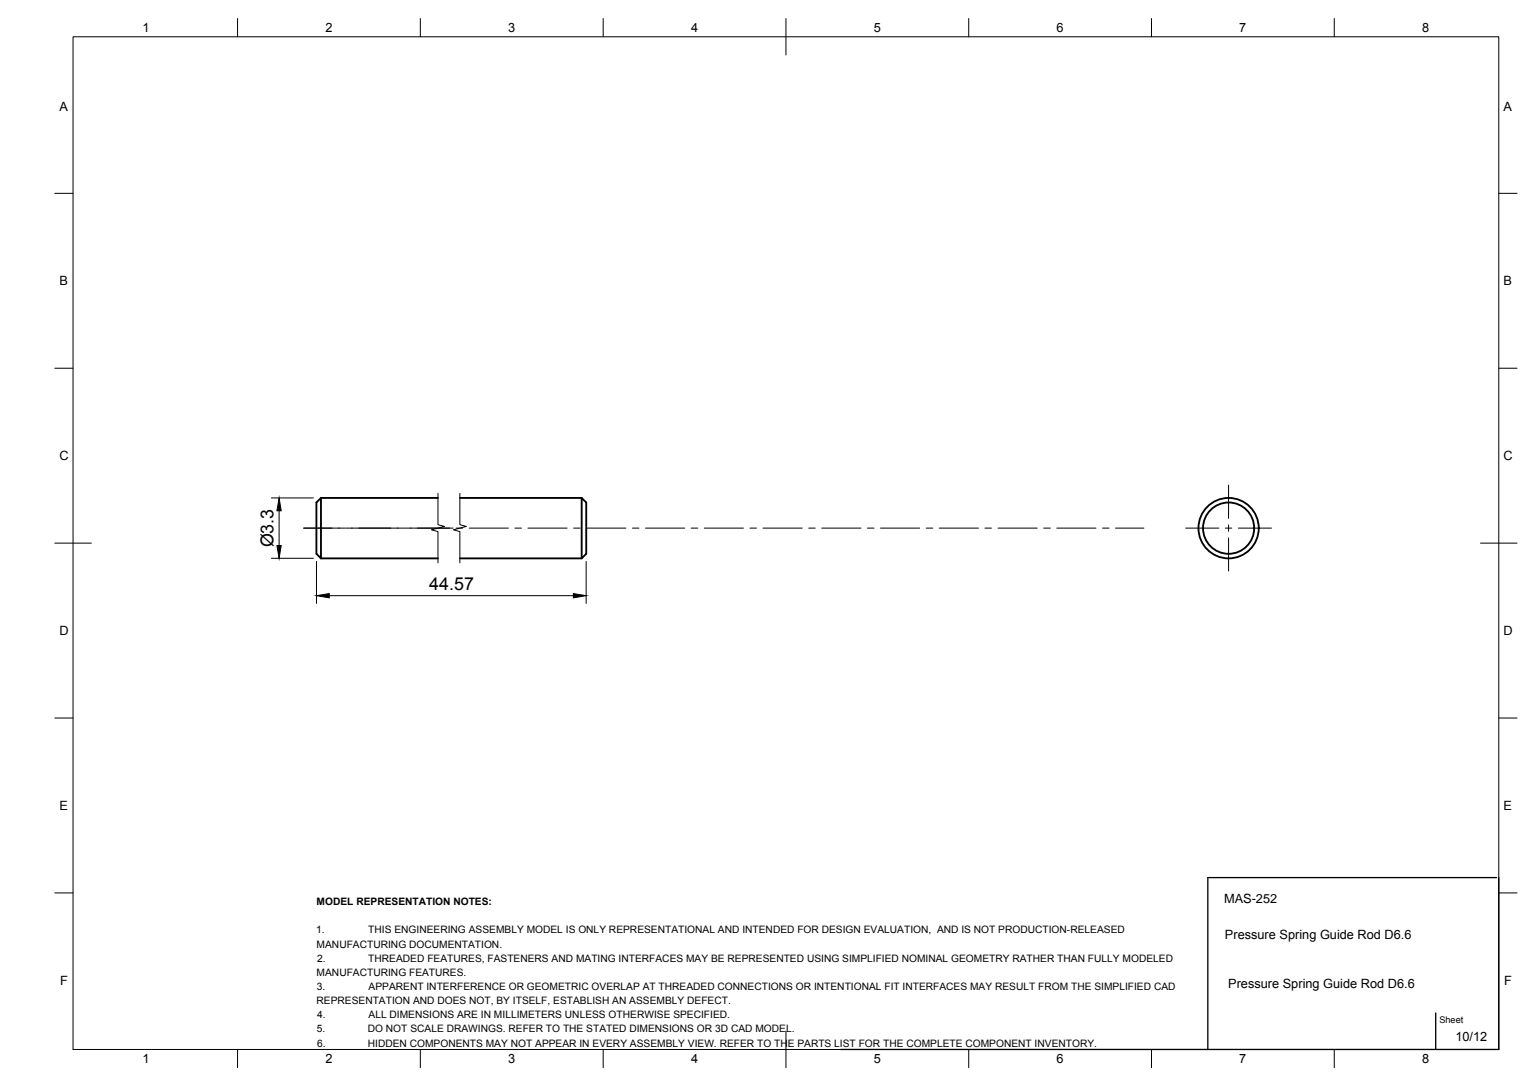
ISO-10303-21;
HEADER;
FILE_DESCRIPTION((''),'2;1');
FILE_NAME('Pressure Spring Guide Rod D6.6.step','2026-10-06T07:01:46+05:00',(''),(''),'','','');
FILE_SCHEMA (('AUTOMOTIVE_DESIGN { 1 0 10303 214 3 1 1 }'));
ENDSEC;
DATA;
#10=MECHANICAL_DESIGN_GEOMETRIC_PRESENTATION_REPRESENTATION('',(#143),#11396);
#99=CONICAL_SURFACE('',#6246,1.525,0.78539816339745) ;
#100=CONICAL_SURFACE('',#6250,1.525,0.78539816339745) ;
#113=SHAPE_REPRESENTATION_RELATIONSHIP('SRR','None',#11460,#128) ;
#128=ADVANCED_BREP_SHAPE_REPRESENTATION('',(#158),#11386) ;
#143=STYLED_ITEM('',(#11544),#158) ;
#158=MANIFOLD_SOLID_BREP('Pressure Spring Guide Rod D6.6',#5574) ;
#466=PLANE('',#6244) ;
#467=PLANE('',#6252) ;
#766=FACE_OUTER_BOUND('',#1130,.T.) ;
#767=FACE_OUTER_BOUND('',#1131,.T.) ;
#768=FACE_OUTER_BOUND('',#1132,.T.) ;
#769=FACE_OUTER_BOUND('',#1133,.T.) ;
#770=FACE_OUTER_BOUND('',#1134,.T.) ;
#1130=EDGE_LOOP('',(#4752)) ;
#1131=EDGE_LOOP('',(#4753,#4754,#4755,#4756)) ;
#1132=EDGE_LOOP('',(#4757,#4758,#4759,#4760)) ;
#1133=EDGE_LOOP('',(#4761,#4762,#4763,#4764)) ;
#1134=EDGE_LOOP('',(#4765)) ;
#1503=LINE('',#10850,#1886) ;
#1504=LINE('',#10854,#1887) ;
#1505=LINE('',#10858,#1888) ;
#1886=VECTOR('',#7693,1.525) ;
#1887=VECTOR('',#7698,1.65) ;
#1888=VECTOR('',#7703,1.525) ;
#2206=CIRCLE('',#6245,1.4) ;
#2207=CIRCLE('',#6247,1.65) ;
#2208=CIRCLE('',#6249,1.65) ;
#2209=CIRCLE('',#6251,1.4) ;
#2635=VERTEX_POINT('',#10845) ;
#2636=VERTEX_POINT('',#10848) ;
#2637=VERTEX_POINT('',#10852) ;
#2638=VERTEX_POINT('',#10856) ;
#3358=EDGE_CURVE('',#2635,#2635,#2206,.T.) ;
#3359=EDGE_CURVE('',#2636,#2636,#2207,.T.) ;
#3360=EDGE_CURVE('',#2636,#2635,#1503,.T.) ;
#3361=EDGE_CURVE('',#2637,#2637,#2208,.T.) ;
#3362=EDGE_CURVE('',#2637,#2636,#1504,.T.) ;
#3363=EDGE_CURVE('',#2638,#2638,#2209,.T.) ;
#3364=EDGE_CURVE('',#2638,#2637,#1505,.T.) ;
#4752=ORIENTED_EDGE('',*,*,#3358,.F.) ;
#4753=ORIENTED_EDGE('',*,*,#3359,.F.) ;
#4754=ORIENTED_EDGE('',*,*,#3360,.T.) ;
#4755=ORIENTED_EDGE('',*,*,#3358,.T.) ;
#4756=ORIENTED_EDGE('',*,*,#3360,.F.) ;
#4757=ORIENTED_EDGE('',*,*,#3361,.F.) ;
#4758=ORIENTED_EDGE('',*,*,#3362,.T.) ;
#4759=ORIENTED_EDGE('',*,*,#3359,.T.) ;
#4760=ORIENTED_EDGE('',*,*,#3362,.F.) ;
#4761=ORIENTED_EDGE('',*,*,#3363,.F.) ;
#4762=ORIENTED_EDGE('',*,*,#3364,.T.) ;
#4763=ORIENTED_EDGE('',*,*,#3361,.T.) ;
#4764=ORIENTED_EDGE('',*,*,#3364,.F.) ;
#4765=ORIENTED_EDGE('',*,*,#3363,.T.) ;
#5208=CYLINDRICAL_SURFACE('',#6248,1.65) ;
#5491=ADVANCED_FACE('',(#766),#466,.T.) ;
#5492=ADVANCED_FACE('',(#767),#99,.T.) ;
#5493=ADVANCED_FACE('',(#768),#5208,.T.) ;
#5494=ADVANCED_FACE('',(#769),#100,.T.) ;
#5495=ADVANCED_FACE('',(#770),#467,.T.) ;
#5574=CLOSED_SHELL('',(#5491,#5492,#5493,#5494,#5495)) ;
#6243=AXIS2_PLACEMENT_3D('',#10843,#7683,#7684) ;
#6244=AXIS2_PLACEMENT_3D('',#10844,#7685,#7686) ;
#6245=AXIS2_PLACEMENT_3D('',#10846,#7687,#7688) ;
#6246=AXIS2_PLACEMENT_3D('',#10847,#7689,#7690) ;
#6247=AXIS2_PLACEMENT_3D('',#10849,#7691,#7692) ;
#6248=AXIS2_PLACEMENT_3D('',#10851,#7694,#7695) ;
#6249=AXIS2_PLACEMENT_3D('',#10853,#7696,#7697) ;
#6250=AXIS2_PLACEMENT_3D('',#10855,#7699,#7700) ;
#6251=AXIS2_PLACEMENT_3D('',#10857,#7701,#7702) ;
#6252=AXIS2_PLACEMENT_3D('',#10859,#7704,#7705) ;
#7683=DIRECTION('axis',(0.,0.,1.)) ;
#7684=DIRECTION('refdir',(1.,0.,0.)) ;
#7685=DIRECTION('center_axis',(0.,0.,-1.)) ;
#7686=DIRECTION('ref_axis',(-1.,0.,0.)) ;
#7687=DIRECTION('center_axis',(0.,0.,1.)) ;
#7688=DIRECTION('ref_axis',(1.,0.,0.)) ;
#7689=DIRECTION('center_axis',(0.,0.,1.)) ;
#7690=DIRECTION('ref_axis',(1.,0.,0.)) ;
#7691=DIRECTION('center_axis',(0.,0.,1.)) ;
#7692=DIRECTION('ref_axis',(1.,0.,0.)) ;
#7693=DIRECTION('',(0.707106781186549,8.65956056235495E-17,-0.707106781186546)) ;
#7694=DIRECTION('center_axis',(0.,0.,1.)) ;
#7695=DIRECTION('ref_axis',(1.,0.,0.)) ;
#7696=DIRECTION('center_axis',(0.,0.,1.)) ;
#7697=DIRECTION('ref_axis',(1.,0.,0.)) ;
#7698=DIRECTION('',(0.,0.,-1.)) ;
#7699=DIRECTION('center_axis',(0.,0.,-1.)) ;
#7700=DIRECTION('ref_axis',(1.,0.,0.)) ;
#7701=DIRECTION('center_axis',(0.,0.,1.)) ;
#7702=DIRECTION('ref_axis',(1.,0.,0.)) ;
#7703=DIRECTION('',(-0.707106781186549,-8.65956056235495E-17,-0.707106781186546)) ;
#7704=DIRECTION('center_axis',(0.,0.,1.)) ;
#7705=DIRECTION('ref_axis',(1.,0.,0.)) ;
#10843=CARTESIAN_POINT('',(0.,0.,0.)) ;
#10844=CARTESIAN_POINT('Origin',(1.875,7.535,-26.18)) ;
#10845=CARTESIAN_POINT('',(-0.924999999999999,7.535,-26.18)) ;
#10846=CARTESIAN_POINT('Origin',(0.475,7.535,-26.18)) ;
#10847=CARTESIAN_POINT('Origin',(0.475,7.535,-26.055)) ;
#10848=CARTESIAN_POINT('',(-1.175,7.535,-25.93)) ;
#10849=CARTESIAN_POINT('Origin',(0.475,7.535,-25.93)) ;
#10850=CARTESIAN_POINT('',(-1.05,7.535,-26.055)) ;
#10851=CARTESIAN_POINT('Origin',(0.475,7.535,-3.895)) ;
#10852=CARTESIAN_POINT('',(-1.175,7.535,18.14)) ;
#10853=CARTESIAN_POINT('Origin',(0.475,7.535,18.14)) ;
#10854=CARTESIAN_POINT('',(-1.175,7.535,-3.895)) ;
#10855=CARTESIAN_POINT('Origin',(0.475,7.535,18.265)) ;
#10856=CARTESIAN_POINT('',(-0.925,7.535,18.39)) ;
#10857=CARTESIAN_POINT('Origin',(0.475,7.535,18.39)) ;
#10858=CARTESIAN_POINT('',(-1.05,7.535,18.265)) ;
#10859=CARTESIAN_POINT('Origin',(0.475,7.535,18.39)) ;
#11369=UNCERTAINTY_MEASURE_WITH_UNIT(LENGTH_MEASURE(0.01),#11397,
'DISTANCE_ACCURACY_VALUE',
'Maximum model space distance between geometric entities at asserted c
onnectivities') ;
#11379=UNCERTAINTY_MEASURE_WITH_UNIT(LENGTH_MEASURE(0.01),#11397,
'DISTANCE_ACCURACY_VALUE',
'Maximum model space distance between geometric entities at asserted c
onnectivities') ;
#11386=(
GEOMETRIC_REPRESENTATION_CONTEXT(3)
GLOBAL_UNCERTAINTY_ASSIGNED_CONTEXT((#11369))
GLOBAL_UNIT_ASSIGNED_CONTEXT((#11397,#11399,#11400))
REPRESENTATION_CONTEXT('','3D')
) ;
#11396=(
GEOMETRIC_REPRESENTATION_CONTEXT(3)
GLOBAL_UNCERTAINTY_ASSIGNED_CONTEXT((#11379))
GLOBAL_UNIT_ASSIGNED_CONTEXT((#11397,#11399,#11400))
REPRESENTATION_CONTEXT('','3D')
) ;
#11397=(
LENGTH_UNIT()
NAMED_UNIT(*)
SI_UNIT(.MILLI.,.METRE.)
) ;
#11399=(
NAMED_UNIT(*)
PLANE_ANGLE_UNIT()
SI_UNIT($,.RADIAN.)
) ;
#11400=(
NAMED_UNIT(*)
SI_UNIT($,.STERADIAN.)
SOLID_ANGLE_UNIT()
) ;
#11407=SHAPE_DEFINITION_REPRESENTATION(#11423,#11460) ;
#11423=PRODUCT_DEFINITION_SHAPE('',$,#11477) ;
#11460=SHAPE_REPRESENTATION('',(#6243),#11386) ;
#11470=PRODUCT_DEFINITION_CONTEXT('part definition',#11520,'design') ;
#11477=PRODUCT_DEFINITION('Pressure Spring Guide Rod D6.6',
'Pressure Spring Guide Rod D6.6',#11493,#11470) ;
#11493=PRODUCT_DEFINITION_FORMATION('',$,#11528) ;
#11520=APPLICATION_CONTEXT(
'Core Data for Automotive Mechanical Design Process') ;
#11521=PRODUCT_CONTEXT('part definition',#11520,'mechanical') ;
#11528=PRODUCT('Pressure Spring Guide Rod D6.6',
'Pressure Spring Guide Rod D6.6',$,(#11521)) ;
#11544=PRESENTATION_STYLE_ASSIGNMENT((#11560)) ;
#11560=SURFACE_STYLE_USAGE(.BOTH.,#11576) ;
#11576=SURFACE_SIDE_STYLE('',(#11592)) ;
#11592=SURFACE_STYLE_FILL_AREA(#11608) ;
#11608=FILL_AREA_STYLE(
'MAS-252 Metallic - Pressure Spring Guide Rod D6.6',(#11624)) ;
#11624=FILL_AREA_STYLE_COLOUR(
'MAS-252 Metallic - Pressure Spring Guide Rod D6.6',#11640) ;
#11640=COLOUR_RGB('MAS-252 Metallic - Pressure Spring Guide Rod D6.6', 0.08235294, 0.09019608, 0.10196078) ;
ENDSEC;
END-ISO-10303-21;
